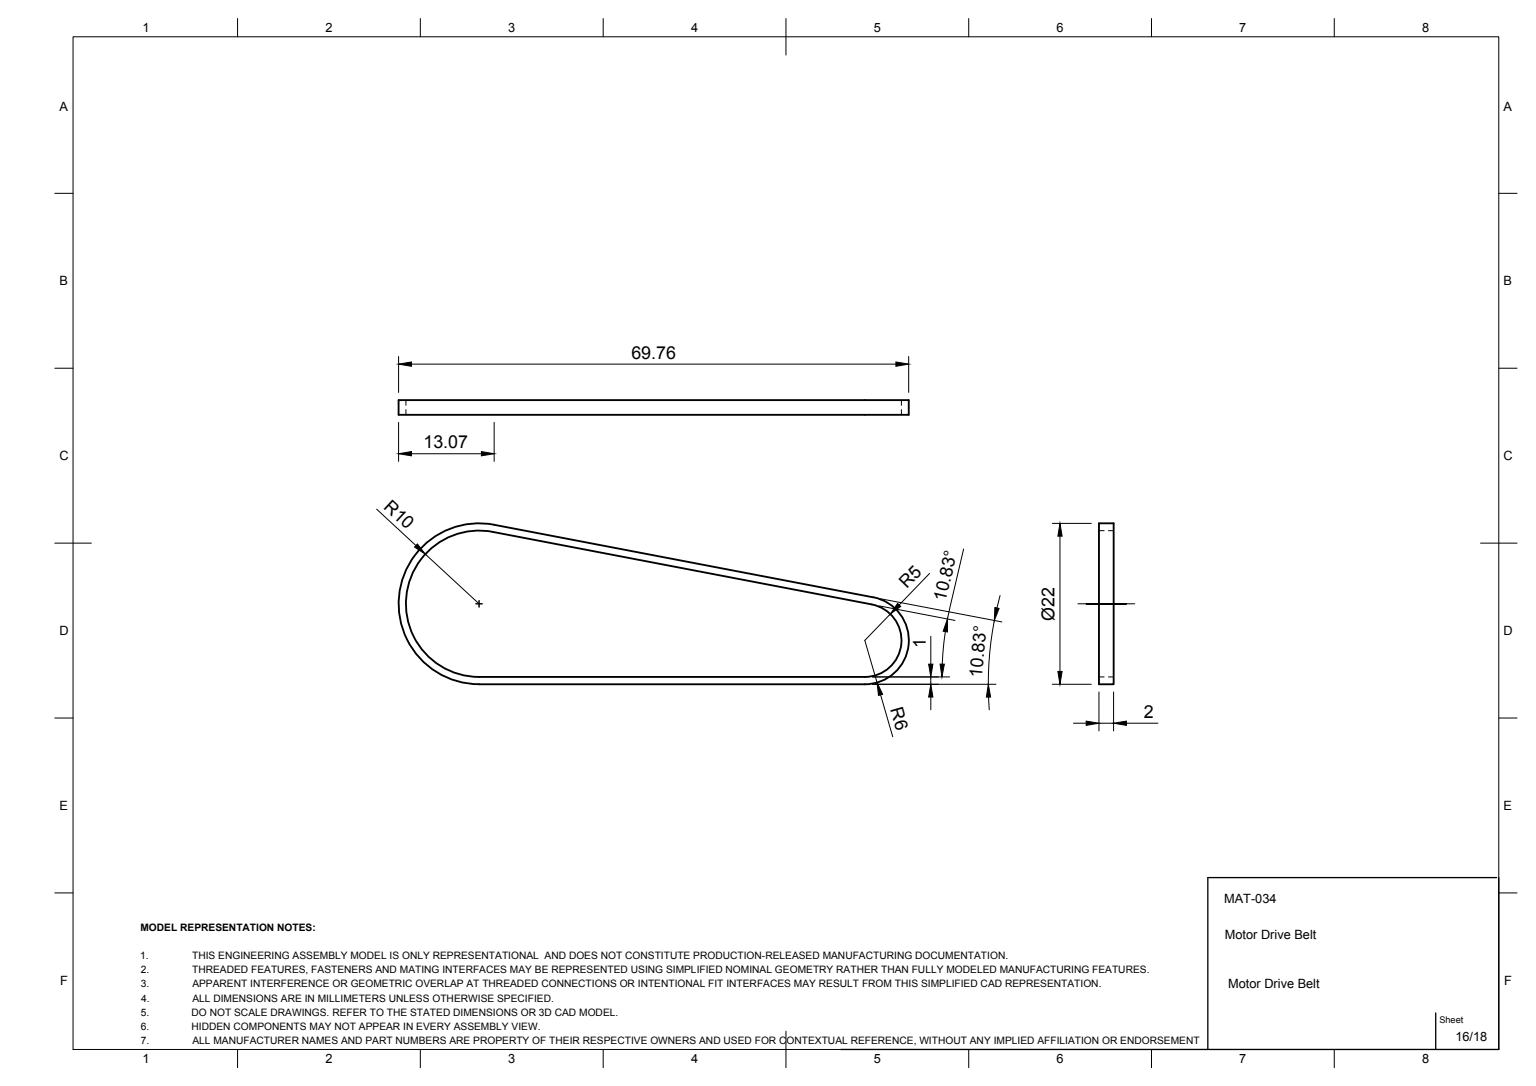
ISO-10303-21;
HEADER;
/* Generated by software containing ST-Developer
 * from STEP Tools, Inc. (www.steptools.com) 
 */

FILE_DESCRIPTION(
/* description */ ('STEP AP214'),
/* implementation_level */ '2;1');

FILE_NAME(
/* name */ 'Motor Drive Belt.step',
/* time_stamp */ '2026-11-14T09:24:36-08:00',
/* author */ (''),
/* organization */ (''),
/* preprocessor_version */ 'ST-DEVELOPER v20.2',
/* originating_system */ 'Autodesk Translation Framework v15.17.0.0',
/* authorisation */ '');

FILE_SCHEMA (('AUTOMOTIVE_DESIGN { 1 0 10303 214 3 1 1 }'));
ENDSEC;

DATA;
#10=MECHANICAL_DESIGN_GEOMETRIC_PRESENTATION_REPRESENTATION('',(#211),#18867);
#179=SHAPE_REPRESENTATION_RELATIONSHIP('SRR','None',#18943,#195);
#195=ADVANCED_BREP_SHAPE_REPRESENTATION('',(#235),#18859);
#211=STYLED_ITEM('',(#19028),#235);
#235=MANIFOLD_SOLID_BREP('Body1',#10966);
#342=FACE_BOUND('',#1692,.T.);
#343=FACE_BOUND('',#1694,.T.);
#552=PLANE('',#11677);
#553=PLANE('',#11680);
#554=PLANE('',#11683);
#555=PLANE('',#11685);
#556=PLANE('',#11686);
#557=PLANE('',#11688);
#1002=FACE_OUTER_BOUND('',#1689,.T.);
#1003=FACE_OUTER_BOUND('',#1690,.T.);
#1004=FACE_OUTER_BOUND('',#1691,.T.);
#1005=FACE_OUTER_BOUND('',#1693,.T.);
#1006=FACE_OUTER_BOUND('',#1695,.T.);
#1007=FACE_OUTER_BOUND('',#1696,.T.);
#1008=FACE_OUTER_BOUND('',#1697,.T.);
#1009=FACE_OUTER_BOUND('',#1698,.T.);
#1010=FACE_OUTER_BOUND('',#1699,.T.);
#1011=FACE_OUTER_BOUND('',#1700,.T.);
#1689=EDGE_LOOP('',(#8460,#8461,#8462,#8463));
#1690=EDGE_LOOP('',(#8464,#8465,#8466,#8467));
#1691=EDGE_LOOP('',(#8468,#8469,#8470,#8471));
#1692=EDGE_LOOP('',(#8472,#8473,#8474,#8475));
#1693=EDGE_LOOP('',(#8476,#8477,#8478,#8479));
#1694=EDGE_LOOP('',(#8480,#8481,#8482,#8483));
#1695=EDGE_LOOP('',(#8484,#8485,#8486,#8487));
#1696=EDGE_LOOP('',(#8488,#8489,#8490,#8491));
#1697=EDGE_LOOP('',(#8492,#8493,#8494,#8495));
#1698=EDGE_LOOP('',(#8496,#8497,#8498,#8499));
#1699=EDGE_LOOP('',(#8500,#8501,#8502,#8503));
#1700=EDGE_LOOP('',(#8504,#8505,#8506,#8507));
#2494=LINE('',#17071,#3508);
#2495=LINE('',#17074,#3509);
#2496=LINE('',#17080,#3510);
#2497=LINE('',#17083,#3511);
#2498=LINE('',#17086,#3512);
#2499=LINE('',#17089,#3513);
#2500=LINE('',#17091,#3514);
#2501=LINE('',#17093,#3515);
#2502=LINE('',#17097,#3516);
#2503=LINE('',#17100,#3517);
#2504=LINE('',#17102,#3518);
#2505=LINE('',#17105,#3519);
#2506=LINE('',#17107,#3520);
#2507=LINE('',#17109,#3521);
#2508=LINE('',#17112,#3522);
#2509=LINE('',#17114,#3523);
#3508=VECTOR('',#13778,1000.);
#3509=VECTOR('',#13781,1000.);
#3510=VECTOR('',#13786,1000.);
#3511=VECTOR('',#13789,1000.);
#3512=VECTOR('',#13792,1000.);
#3513=VECTOR('',#13795,1000.);
#3514=VECTOR('',#13796,1000.);
#3515=VECTOR('',#13797,1000.);
#3516=VECTOR('',#13802,1000.);
#3517=VECTOR('',#13805,1000.);
#3518=VECTOR('',#13806,1000.);
#3519=VECTOR('',#13809,1000.);
#3520=VECTOR('',#13812,1000.);
#3521=VECTOR('',#13815,1000.);
#3522=VECTOR('',#13820,1000.);
#3523=VECTOR('',#13823,1000.);
#4296=CIRCLE('',#11672,5.);
#4297=CIRCLE('',#11673,5.);
#4298=CIRCLE('',#11675,6.);
#4299=CIRCLE('',#11676,6.);
#4300=CIRCLE('',#11678,11.);
#4301=CIRCLE('',#11679,10.);
#4302=CIRCLE('',#11681,11.);
#4303=CIRCLE('',#11682,10.);
#5020=VERTEX_POINT('',#17067);
#5021=VERTEX_POINT('',#17068);
#5022=VERTEX_POINT('',#17070);
#5023=VERTEX_POINT('',#17072);
#5024=VERTEX_POINT('',#17076);
#5025=VERTEX_POINT('',#17077);
#5026=VERTEX_POINT('',#17079);
#5027=VERTEX_POINT('',#17081);
#5028=VERTEX_POINT('',#17085);
#5029=VERTEX_POINT('',#17087);
#5030=VERTEX_POINT('',#17090);
#5031=VERTEX_POINT('',#17092);
#5032=VERTEX_POINT('',#17096);
#5033=VERTEX_POINT('',#17098);
#5034=VERTEX_POINT('',#17101);
#5035=VERTEX_POINT('',#17103);
#6263=EDGE_CURVE('',#5020,#5021,#4296,.T.);
#6264=EDGE_CURVE('',#5021,#5022,#2494,.T.);
#6265=EDGE_CURVE('',#5023,#5022,#4297,.T.);
#6266=EDGE_CURVE('',#5020,#5023,#2495,.T.);
#6267=EDGE_CURVE('',#5024,#5025,#4298,.T.);
#6268=EDGE_CURVE('',#5024,#5026,#2496,.T.);
#6269=EDGE_CURVE('',#5026,#5027,#4299,.T.);
#6270=EDGE_CURVE('',#5025,#5027,#2497,.T.);
#6271=EDGE_CURVE('',#5025,#5028,#2498,.T.);
#6272=EDGE_CURVE('',#5028,#5029,#4300,.T.);
#6273=EDGE_CURVE('',#5029,#5024,#2499,.T.);
#6274=EDGE_CURVE('',#5021,#5030,#2500,.T.);
#6275=EDGE_CURVE('',#5031,#5020,#2501,.T.);
#6276=EDGE_CURVE('',#5030,#5031,#4301,.T.);
#6277=EDGE_CURVE('',#5032,#5026,#2502,.T.);
#6278=EDGE_CURVE('',#5033,#5032,#4302,.T.);
#6279=EDGE_CURVE('',#5027,#5033,#2503,.T.);
#6280=EDGE_CURVE('',#5022,#5034,#2504,.T.);
#6281=EDGE_CURVE('',#5034,#5035,#4303,.T.);
#6282=EDGE_CURVE('',#5035,#5023,#2505,.T.);
#6283=EDGE_CURVE('',#5028,#5033,#2506,.T.);
#6284=EDGE_CURVE('',#5029,#5032,#2507,.T.);
#6285=EDGE_CURVE('',#5030,#5034,#2508,.T.);
#6286=EDGE_CURVE('',#5031,#5035,#2509,.T.);
#8460=ORIENTED_EDGE('',*,*,#6263,.T.);
#8461=ORIENTED_EDGE('',*,*,#6264,.T.);
#8462=ORIENTED_EDGE('',*,*,#6265,.F.);
#8463=ORIENTED_EDGE('',*,*,#6266,.F.);
#8464=ORIENTED_EDGE('',*,*,#6267,.F.);
#8465=ORIENTED_EDGE('',*,*,#6268,.T.);
#8466=ORIENTED_EDGE('',*,*,#6269,.T.);
#8467=ORIENTED_EDGE('',*,*,#6270,.F.);
#8468=ORIENTED_EDGE('',*,*,#6267,.T.);
#8469=ORIENTED_EDGE('',*,*,#6271,.T.);
#8470=ORIENTED_EDGE('',*,*,#6272,.T.);
#8471=ORIENTED_EDGE('',*,*,#6273,.T.);
#8472=ORIENTED_EDGE('',*,*,#6274,.F.);
#8473=ORIENTED_EDGE('',*,*,#6263,.F.);
#8474=ORIENTED_EDGE('',*,*,#6275,.F.);
#8475=ORIENTED_EDGE('',*,*,#6276,.F.);
#8476=ORIENTED_EDGE('',*,*,#6269,.F.);
#8477=ORIENTED_EDGE('',*,*,#6277,.F.);
#8478=ORIENTED_EDGE('',*,*,#6278,.F.);
#8479=ORIENTED_EDGE('',*,*,#6279,.F.);
#8480=ORIENTED_EDGE('',*,*,#6265,.T.);
#8481=ORIENTED_EDGE('',*,*,#6280,.T.);
#8482=ORIENTED_EDGE('',*,*,#6281,.T.);
#8483=ORIENTED_EDGE('',*,*,#6282,.T.);
#8484=ORIENTED_EDGE('',*,*,#6279,.T.);
#8485=ORIENTED_EDGE('',*,*,#6283,.F.);
#8486=ORIENTED_EDGE('',*,*,#6271,.F.);
#8487=ORIENTED_EDGE('',*,*,#6270,.T.);
#8488=ORIENTED_EDGE('',*,*,#6278,.T.);
#8489=ORIENTED_EDGE('',*,*,#6284,.F.);
#8490=ORIENTED_EDGE('',*,*,#6272,.F.);
#8491=ORIENTED_EDGE('',*,*,#6283,.T.);
#8492=ORIENTED_EDGE('',*,*,#6277,.T.);
#8493=ORIENTED_EDGE('',*,*,#6268,.F.);
#8494=ORIENTED_EDGE('',*,*,#6273,.F.);
#8495=ORIENTED_EDGE('',*,*,#6284,.T.);
#8496=ORIENTED_EDGE('',*,*,#6280,.F.);
#8497=ORIENTED_EDGE('',*,*,#6264,.F.);
#8498=ORIENTED_EDGE('',*,*,#6274,.T.);
#8499=ORIENTED_EDGE('',*,*,#6285,.T.);
#8500=ORIENTED_EDGE('',*,*,#6281,.F.);
#8501=ORIENTED_EDGE('',*,*,#6285,.F.);
#8502=ORIENTED_EDGE('',*,*,#6276,.T.);
#8503=ORIENTED_EDGE('',*,*,#6286,.T.);
#8504=ORIENTED_EDGE('',*,*,#6282,.F.);
#8505=ORIENTED_EDGE('',*,*,#6286,.F.);
#8506=ORIENTED_EDGE('',*,*,#6275,.T.);
#8507=ORIENTED_EDGE('',*,*,#6266,.T.);
#10245=CYLINDRICAL_SURFACE('',#11671,5.);
#10246=CYLINDRICAL_SURFACE('',#11674,6.);
#10247=CYLINDRICAL_SURFACE('',#11684,11.);
#10248=CYLINDRICAL_SURFACE('',#11687,10.);
#10639=ADVANCED_FACE('',(#1002),#10245,.F.);
#10640=ADVANCED_FACE('',(#1003),#10246,.T.);
#10641=ADVANCED_FACE('',(#1004,#342),#552,.T.);
#10642=ADVANCED_FACE('',(#1005,#343),#553,.F.);
#10643=ADVANCED_FACE('',(#1006),#554,.F.);
#10644=ADVANCED_FACE('',(#1007),#10247,.T.);
#10645=ADVANCED_FACE('',(#1008),#555,.F.);
#10646=ADVANCED_FACE('',(#1009),#556,.T.);
#10647=ADVANCED_FACE('',(#1010),#10248,.F.);
#10648=ADVANCED_FACE('',(#1011),#557,.T.);
#10966=CLOSED_SHELL('',(#10639,#10640,#10641,#10642,#10643,#10644,#10645,
#10646,#10647,#10648));
#11670=AXIS2_PLACEMENT_3D('',#17065,#13772,#13773);
#11671=AXIS2_PLACEMENT_3D('',#17066,#13774,#13775);
#11672=AXIS2_PLACEMENT_3D('',#17069,#13776,#13777);
#11673=AXIS2_PLACEMENT_3D('',#17073,#13779,#13780);
#11674=AXIS2_PLACEMENT_3D('',#17075,#13782,#13783);
#11675=AXIS2_PLACEMENT_3D('',#17078,#13784,#13785);
#11676=AXIS2_PLACEMENT_3D('',#17082,#13787,#13788);
#11677=AXIS2_PLACEMENT_3D('',#17084,#13790,#13791);
#11678=AXIS2_PLACEMENT_3D('',#17088,#13793,#13794);
#11679=AXIS2_PLACEMENT_3D('',#17094,#13798,#13799);
#11680=AXIS2_PLACEMENT_3D('',#17095,#13800,#13801);
#11681=AXIS2_PLACEMENT_3D('',#17099,#13803,#13804);
#11682=AXIS2_PLACEMENT_3D('',#17104,#13807,#13808);
#11683=AXIS2_PLACEMENT_3D('',#17106,#13810,#13811);
#11684=AXIS2_PLACEMENT_3D('',#17108,#13813,#13814);
#11685=AXIS2_PLACEMENT_3D('',#17110,#13816,#13817);
#11686=AXIS2_PLACEMENT_3D('',#17111,#13818,#13819);
#11687=AXIS2_PLACEMENT_3D('',#17113,#13821,#13822);
#11688=AXIS2_PLACEMENT_3D('',#17115,#13824,#13825);
#13772=DIRECTION('axis',(0.,0.,1.));
#13773=DIRECTION('refdir',(1.,0.,0.));
#13774=DIRECTION('center_axis',(0.,0.,-1.));
#13775=DIRECTION('ref_axis',(-1.,0.,0.));
#13776=DIRECTION('center_axis',(0.,0.,1.));
#13777=DIRECTION('ref_axis',(1.,0.,0.));
#13778=DIRECTION('',(0.,0.,-1.));
#13779=DIRECTION('center_axis',(0.,0.,1.));
#13780=DIRECTION('ref_axis',(1.,0.,0.));
#13781=DIRECTION('',(0.,0.,-1.));
#13782=DIRECTION('center_axis',(0.,0.,-1.));
#13783=DIRECTION('ref_axis',(-1.,0.,0.));
#13784=DIRECTION('center_axis',(0.,0.,1.));
#13785=DIRECTION('ref_axis',(1.,0.,0.));
#13786=DIRECTION('',(0.,0.,-1.));
#13787=DIRECTION('center_axis',(0.,0.,1.));
#13788=DIRECTION('ref_axis',(1.,0.,0.));
#13789=DIRECTION('',(0.,0.,-1.));
#13790=DIRECTION('center_axis',(0.,0.,1.));
#13791=DIRECTION('ref_axis',(1.,0.,0.));
#13792=DIRECTION('',(0.995540072322484,-0.0943396226415094,0.));
#13793=DIRECTION('center_axis',(0.,0.,1.));
#13794=DIRECTION('ref_axis',(1.,0.,0.));
#13795=DIRECTION('',(-0.995540072322484,-0.0943396226415094,0.));
#13796=DIRECTION('',(0.995540072322484,-0.0943396226415095,0.));
#13797=DIRECTION('',(-0.995540072322484,-0.0943396226415095,0.));
#13798=DIRECTION('center_axis',(0.,0.,1.));
#13799=DIRECTION('ref_axis',(1.,0.,0.));
#13800=DIRECTION('center_axis',(0.,0.,1.));
#13801=DIRECTION('ref_axis',(1.,0.,0.));
#13802=DIRECTION('',(-0.995540072322484,-0.0943396226415094,0.));
#13803=DIRECTION('center_axis',(0.,0.,1.));
#13804=DIRECTION('ref_axis',(1.,0.,0.));
#13805=DIRECTION('',(0.995540072322484,-0.0943396226415094,0.));
#13806=DIRECTION('',(0.995540072322484,-0.0943396226415095,0.));
#13807=DIRECTION('center_axis',(0.,0.,1.));
#13808=DIRECTION('ref_axis',(1.,0.,0.));
#13809=DIRECTION('',(-0.995540072322484,-0.0943396226415095,0.));
#13810=DIRECTION('center_axis',(0.0943396226415094,0.995540072322485,0.));
#13811=DIRECTION('ref_axis',(-0.995540072322485,0.0943396226415094,0.));
#13812=DIRECTION('',(0.,0.,-1.));
#13813=DIRECTION('center_axis',(0.,0.,-1.));
#13814=DIRECTION('ref_axis',(1.,-3.21624529935327E-16,0.));
#13815=DIRECTION('',(0.,0.,-1.));
#13816=DIRECTION('center_axis',(0.0943396226415095,-0.995540072322485,0.));
#13817=DIRECTION('ref_axis',(0.995540072322485,0.0943396226415095,0.));
#13818=DIRECTION('center_axis',(0.0943396226415095,0.995540072322485,0.));
#13819=DIRECTION('ref_axis',(-0.995540072322485,0.0943396226415095,0.));
#13820=DIRECTION('',(0.,0.,-1.));
#13821=DIRECTION('center_axis',(0.,0.,-1.));
#13822=DIRECTION('ref_axis',(1.,1.22464679914735E-16,0.));
#13823=DIRECTION('',(0.,0.,-1.));
#13824=DIRECTION('center_axis',(0.0943396226415095,-0.995540072322485,0.));
#13825=DIRECTION('ref_axis',(0.995540072322485,0.0943396226415095,0.));
#17065=CARTESIAN_POINT('',(0.,0.,0.));
#17066=CARTESIAN_POINT('Origin',(-53.,0.,1.));
#17067=CARTESIAN_POINT('',(-53.4716981132075,4.97770036161242,1.));
#17068=CARTESIAN_POINT('',(-53.4716981132075,-4.97770036161242,1.));
#17069=CARTESIAN_POINT('Origin',(-53.,0.,1.));
#17070=CARTESIAN_POINT('',(-53.4716981132075,-4.97770036161242,-1.));
#17071=CARTESIAN_POINT('',(-53.4716981132075,-4.97770036161242,1.));
#17072=CARTESIAN_POINT('',(-53.4716981132075,4.97770036161242,-1.));
#17073=CARTESIAN_POINT('Origin',(-53.,0.,-1.));
#17074=CARTESIAN_POINT('',(-53.4716981132075,4.97770036161242,1.));
#17075=CARTESIAN_POINT('Origin',(-53.,0.,1.));
#17076=CARTESIAN_POINT('',(-53.5660377358491,5.97324043393491,1.));
#17077=CARTESIAN_POINT('',(-53.5660377358491,-5.97324043393491,1.));
#17078=CARTESIAN_POINT('Origin',(-53.,0.,1.));
#17079=CARTESIAN_POINT('',(-53.5660377358491,5.97324043393491,-1.));
#17080=CARTESIAN_POINT('',(-53.5660377358491,5.97324043393491,1.));
#17081=CARTESIAN_POINT('',(-53.5660377358491,-5.97324043393491,-1.));
#17082=CARTESIAN_POINT('Origin',(-53.,0.,-1.));
#17083=CARTESIAN_POINT('',(-53.5660377358491,-5.97324043393491,1.));
#17084=CARTESIAN_POINT('Origin',(-53.,0.,1.));
#17085=CARTESIAN_POINT('',(-1.0377358490566,-10.9509407955473,1.));
#17086=CARTESIAN_POINT('',(-1.0377358490566,-10.9509407955473,1.));
#17087=CARTESIAN_POINT('',(-1.03773584905659,10.9509407955473,1.));
#17088=CARTESIAN_POINT('Origin',(0.,0.,1.));
#17089=CARTESIAN_POINT('',(-53.5660377358491,5.97324043393491,1.));
#17090=CARTESIAN_POINT('',(-0.943396226415095,-9.95540072322485,1.));
#17091=CARTESIAN_POINT('',(-0.943396226415095,-9.95540072322485,1.));
#17092=CARTESIAN_POINT('',(-0.943396226415094,9.95540072322485,1.));
#17093=CARTESIAN_POINT('',(-53.4716981132075,4.97770036161242,1.));
#17094=CARTESIAN_POINT('Origin',(0.,0.,1.));
#17095=CARTESIAN_POINT('Origin',(-53.,0.,-1.));
#17096=CARTESIAN_POINT('',(-1.03773584905659,10.9509407955473,-1.));
#17097=CARTESIAN_POINT('',(-53.5660377358491,5.97324043393491,-1.));
#17098=CARTESIAN_POINT('',(-1.0377358490566,-10.9509407955473,-1.));
#17099=CARTESIAN_POINT('Origin',(0.,0.,-1.));
#17100=CARTESIAN_POINT('',(-1.0377358490566,-10.9509407955473,-1.));
#17101=CARTESIAN_POINT('',(-0.943396226415095,-9.95540072322485,-1.));
#17102=CARTESIAN_POINT('',(-0.943396226415095,-9.95540072322485,-1.));
#17103=CARTESIAN_POINT('',(-0.943396226415092,9.95540072322485,-1.));
#17104=CARTESIAN_POINT('Origin',(0.,0.,-1.));
#17105=CARTESIAN_POINT('',(-53.4716981132075,4.97770036161242,-1.));
#17106=CARTESIAN_POINT('Origin',(-1.0377358490566,-10.9509407955473,1.));
#17107=CARTESIAN_POINT('',(-1.0377358490566,-10.9509407955473,1.));
#17108=CARTESIAN_POINT('Origin',(0.,0.,1.));
#17109=CARTESIAN_POINT('',(-1.03773584905659,10.9509407955473,1.));
#17110=CARTESIAN_POINT('Origin',(-53.5660377358491,5.97324043393491,1.));
#17111=CARTESIAN_POINT('Origin',(-0.943396226415095,-9.95540072322485,1.));
#17112=CARTESIAN_POINT('',(-0.943396226415095,-9.95540072322485,1.));
#17113=CARTESIAN_POINT('Origin',(0.,0.,1.));
#17114=CARTESIAN_POINT('',(-0.943396226415092,9.95540072322485,1.));
#17115=CARTESIAN_POINT('Origin',(-53.4716981132075,4.97770036161242,1.));
#18841=UNCERTAINTY_MEASURE_WITH_UNIT(LENGTH_MEASURE(0.01),#18868,
'DISTANCE_ACCURACY_VALUE',
'Maximum model space distance between geometric entities at asserted c
onnectivities');
#18849=UNCERTAINTY_MEASURE_WITH_UNIT(LENGTH_MEASURE(0.01),#18868,
'DISTANCE_ACCURACY_VALUE',
'Maximum model space distance between geometric entities at asserted c
onnectivities');
#18859=(
GEOMETRIC_REPRESENTATION_CONTEXT(3)
GLOBAL_UNCERTAINTY_ASSIGNED_CONTEXT((#18841))
GLOBAL_UNIT_ASSIGNED_CONTEXT((#18868,#18870,#18871))
REPRESENTATION_CONTEXT('','3D')
);
#18867=(
GEOMETRIC_REPRESENTATION_CONTEXT(3)
GLOBAL_UNCERTAINTY_ASSIGNED_CONTEXT((#18849))
GLOBAL_UNIT_ASSIGNED_CONTEXT((#18868,#18870,#18871))
REPRESENTATION_CONTEXT('','3D')
);
#18868=(
LENGTH_UNIT()
NAMED_UNIT(*)
SI_UNIT(.MILLI.,.METRE.)
);
#18870=(
NAMED_UNIT(*)
PLANE_ANGLE_UNIT()
SI_UNIT($,.RADIAN.)
);
#18871=(
NAMED_UNIT(*)
SI_UNIT($,.STERADIAN.)
SOLID_ANGLE_UNIT()
);
#18881=SHAPE_DEFINITION_REPRESENTATION(#18898,#18943);
#18898=PRODUCT_DEFINITION_SHAPE('',$,#18961);
#18943=SHAPE_REPRESENTATION('',(#11670),#18859);
#18951=PRODUCT_DEFINITION_CONTEXT('part definition',#19004,'design');
#18961=PRODUCT_DEFINITION('Motor Drive Belt','Motor Drive Belt',#18978,
#18951);
#18978=PRODUCT_DEFINITION_FORMATION('',$,#19015);
#19004=APPLICATION_CONTEXT(
'Core Data for Automotive Mechanical Design Process');
#19005=PRODUCT_CONTEXT('part definition',#19004,'mechanical');
#19015=PRODUCT('Motor Drive Belt','Motor Drive Belt',$,(#19005));
#19028=PRESENTATION_STYLE_ASSIGNMENT((#19034));
#19034=SURFACE_STYLE_USAGE(.BOTH.,#19040);
#19040=SURFACE_SIDE_STYLE('',(#19046));
#19046=SURFACE_STYLE_FILL_AREA(#19052);
#19052=FILL_AREA_STYLE('Opaque(31,36,43)',(#19058));
#19058=FILL_AREA_STYLE_COLOUR('Opaque(31,36,43)',#19064);
#19064=COLOUR_RGB('Opaque(31,36,43)',0.12156862745098,0.141176470588235,
0.168627450980392);
ENDSEC;
END-ISO-10303-21;
